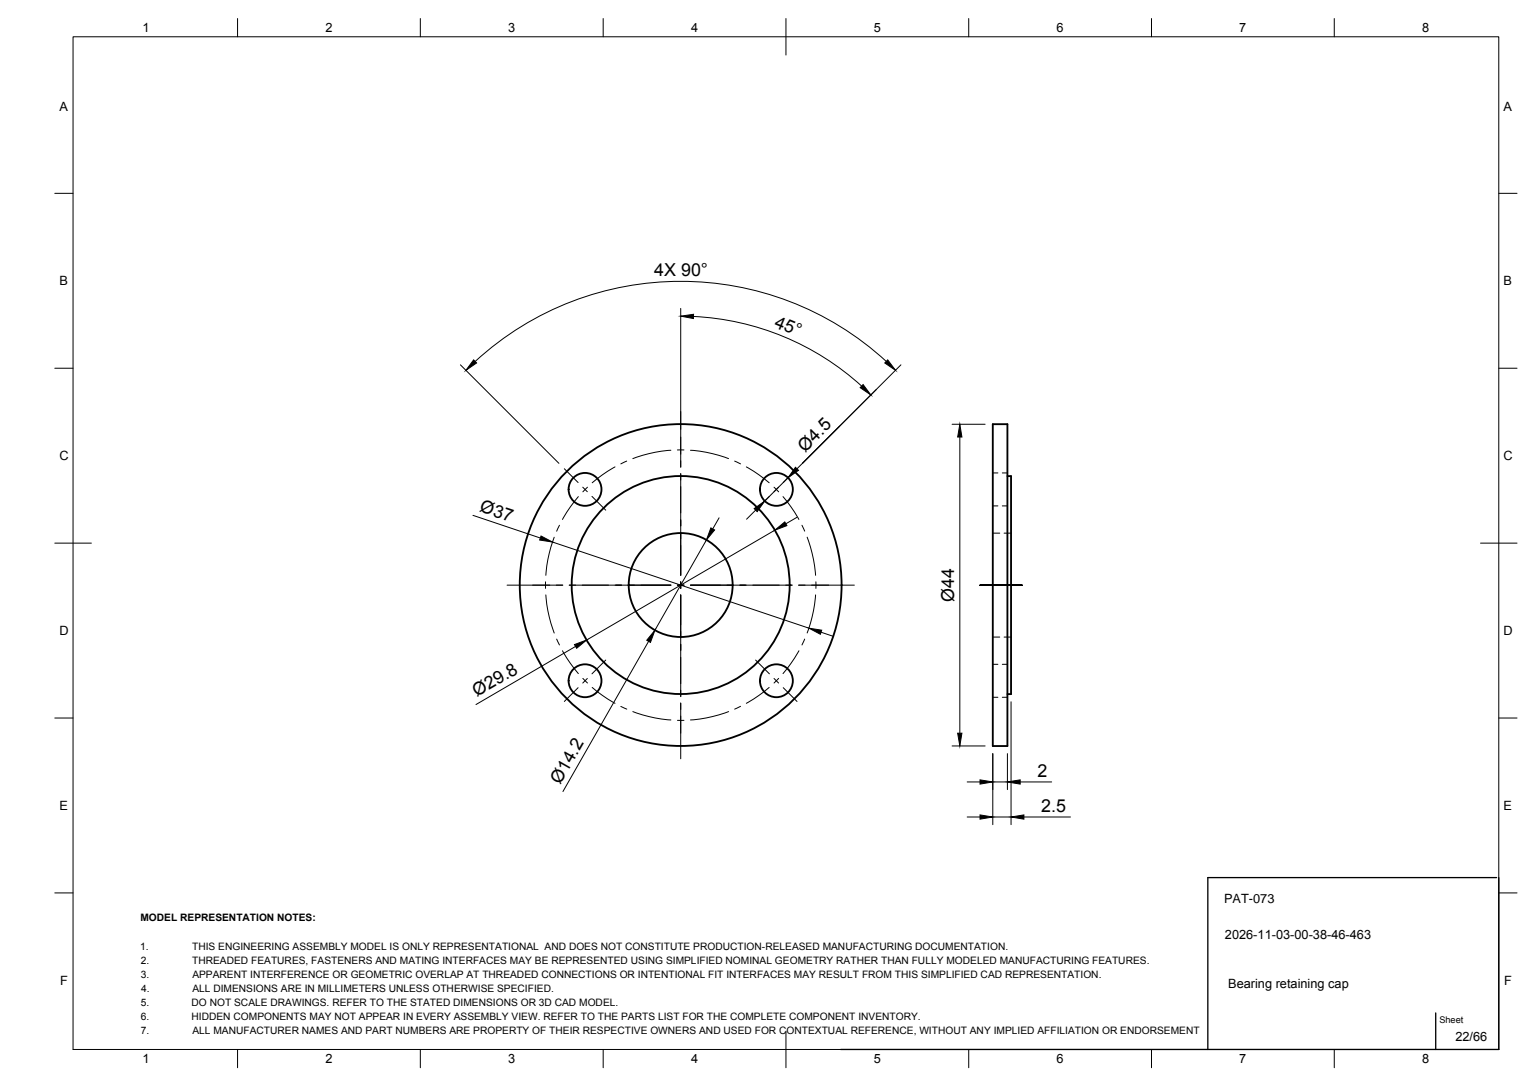
ISO-10303-21;
HEADER;
/* Generated by software containing ST-Developer
 * from STEP Tools, Inc. (www.steptools.com) 
 */

FILE_DESCRIPTION(
/* description */ ('Manual piston pump'),
/* implementation_level */ '2;1');

FILE_NAME(
/* name */ 'Bearing retaining cap.step',
/* time_stamp */ '2026-11-02T16:54:23-08:00',
/* author */ (''),
/* organization */ (''),
/* preprocessor_version */ 'ST-DEVELOPER v20.2',
/* originating_system */ 'Autodesk Translation Framework v15.17.0.0',
/* authorisation */ '');

FILE_SCHEMA (('AUTOMOTIVE_DESIGN { 1 0 10303 214 3 1 1 }'));
ENDSEC;

DATA;
#10=MECHANICAL_DESIGN_GEOMETRIC_PRESENTATION_REPRESENTATION('',(#708),#19043);
#582=SHAPE_REPRESENTATION_RELATIONSHIP('SRR','None',#19328,#645);
#645=ADVANCED_BREP_SHAPE_REPRESENTATION('',(#779),#18995);
#708=STYLED_ITEM('',(#19664),#779);
#779=MANIFOLD_SOLID_BREP('Body1',#9493);
#917=FACE_BOUND('',#2156,.T.);
#918=FACE_BOUND('',#2160,.T.);
#919=FACE_BOUND('',#2161,.T.);
#920=FACE_BOUND('',#2162,.T.);
#921=FACE_BOUND('',#2163,.T.);
#922=FACE_BOUND('',#2164,.T.);
#923=FACE_BOUND('',#2166,.T.);
#924=FACE_BOUND('',#2167,.T.);
#925=FACE_BOUND('',#2168,.T.);
#926=FACE_BOUND('',#2169,.T.);
#927=FACE_BOUND('',#2170,.T.);
#1164=CYLINDRICAL_SURFACE('',#10616,0.225);
#1165=CYLINDRICAL_SURFACE('',#10619,0.225);
#1166=CYLINDRICAL_SURFACE('',#10622,0.225);
#1167=CYLINDRICAL_SURFACE('',#10625,0.225);
#1168=CYLINDRICAL_SURFACE('',#10628,1.49);
#1169=CYLINDRICAL_SURFACE('',#10633,0.710000000000001);
#1170=CYLINDRICAL_SURFACE('',#10635,2.2);
#1485=FACE_OUTER_BOUND('',#2150,.T.);
#1486=FACE_OUTER_BOUND('',#2151,.T.);
#1487=FACE_OUTER_BOUND('',#2152,.T.);
#1488=FACE_OUTER_BOUND('',#2153,.T.);
#1489=FACE_OUTER_BOUND('',#2154,.T.);
#1490=FACE_OUTER_BOUND('',#2155,.T.);
#1491=FACE_OUTER_BOUND('',#2157,.T.);
#1492=FACE_OUTER_BOUND('',#2158,.T.);
#1493=FACE_OUTER_BOUND('',#2159,.T.);
#1494=FACE_OUTER_BOUND('',#2165,.T.);
#2150=EDGE_LOOP('',(#7063,#7064,#7065,#7066));
#2151=EDGE_LOOP('',(#7067,#7068,#7069,#7070));
#2152=EDGE_LOOP('',(#7071,#7072,#7073,#7074));
#2153=EDGE_LOOP('',(#7075,#7076,#7077,#7078));
#2154=EDGE_LOOP('',(#7079,#7080,#7081,#7082));
#2155=EDGE_LOOP('',(#7083));
#2156=EDGE_LOOP('',(#7084));
#2157=EDGE_LOOP('',(#7085,#7086,#7087,#7088));
#2158=EDGE_LOOP('',(#7089,#7090,#7091,#7092));
#2159=EDGE_LOOP('',(#7093));
#2160=EDGE_LOOP('',(#7094));
#2161=EDGE_LOOP('',(#7095));
#2162=EDGE_LOOP('',(#7096));
#2163=EDGE_LOOP('',(#7097));
#2164=EDGE_LOOP('',(#7098));
#2165=EDGE_LOOP('',(#7099));
#2166=EDGE_LOOP('',(#7100));
#2167=EDGE_LOOP('',(#7101));
#2168=EDGE_LOOP('',(#7102));
#2169=EDGE_LOOP('',(#7103));
#2170=EDGE_LOOP('',(#7104));
#2820=CIRCLE('',#10617,0.225);
#2821=CIRCLE('',#10618,0.225);
#2822=CIRCLE('',#10620,0.225);
#2823=CIRCLE('',#10621,0.225);
#2824=CIRCLE('',#10623,0.225);
#2825=CIRCLE('',#10624,0.225);
#2826=CIRCLE('',#10626,0.225);
#2827=CIRCLE('',#10627,0.225);
#2828=CIRCLE('',#10629,1.49);
#2829=CIRCLE('',#10630,1.49);
#2830=CIRCLE('',#10632,0.710000000000001);
#2831=CIRCLE('',#10634,0.710000000000001);
#2832=CIRCLE('',#10636,2.2);
#2833=CIRCLE('',#10637,2.2);
#3370=LINE('',#15553,#3974);
#3371=LINE('',#15559,#3975);
#3372=LINE('',#15565,#3976);
#3373=LINE('',#15571,#3977);
#3374=LINE('',#15577,#3978);
#3375=LINE('',#15584,#3979);
#3376=LINE('',#15590,#3980);
#3974=VECTOR('',#12468,0.225);
#3975=VECTOR('',#12475,0.225);
#3976=VECTOR('',#12482,0.225);
#3977=VECTOR('',#12489,0.225);
#3978=VECTOR('',#12496,1.49);
#3979=VECTOR('',#12505,0.710000000000001);
#3980=VECTOR('',#12512,2.2);
#4615=VERTEX_POINT('',#15550);
#4616=VERTEX_POINT('',#15552);
#4617=VERTEX_POINT('',#15556);
#4618=VERTEX_POINT('',#15558);
#4619=VERTEX_POINT('',#15562);
#4620=VERTEX_POINT('',#15564);
#4621=VERTEX_POINT('',#15568);
#4622=VERTEX_POINT('',#15570);
#4623=VERTEX_POINT('',#15574);
#4624=VERTEX_POINT('',#15576);
#4625=VERTEX_POINT('',#15580);
#4626=VERTEX_POINT('',#15583);
#4627=VERTEX_POINT('',#15587);
#4628=VERTEX_POINT('',#15589);
#5518=EDGE_CURVE('',#4615,#4615,#2820,.T.);
#5519=EDGE_CURVE('',#4615,#4616,#3370,.T.);
#5520=EDGE_CURVE('',#4616,#4616,#2821,.T.);
#5521=EDGE_CURVE('',#4617,#4617,#2822,.T.);
#5522=EDGE_CURVE('',#4617,#4618,#3371,.T.);
#5523=EDGE_CURVE('',#4618,#4618,#2823,.T.);
#5524=EDGE_CURVE('',#4619,#4619,#2824,.T.);
#5525=EDGE_CURVE('',#4619,#4620,#3372,.T.);
#5526=EDGE_CURVE('',#4620,#4620,#2825,.T.);
#5527=EDGE_CURVE('',#4621,#4621,#2826,.T.);
#5528=EDGE_CURVE('',#4621,#4622,#3373,.T.);
#5529=EDGE_CURVE('',#4622,#4622,#2827,.T.);
#5530=EDGE_CURVE('',#4623,#4623,#2828,.T.);
#5531=EDGE_CURVE('',#4623,#4624,#3374,.T.);
#5532=EDGE_CURVE('',#4624,#4624,#2829,.T.);
#5533=EDGE_CURVE('',#4625,#4625,#2830,.T.);
#5534=EDGE_CURVE('',#4625,#4626,#3375,.T.);
#5535=EDGE_CURVE('',#4626,#4626,#2831,.T.);
#5536=EDGE_CURVE('',#4627,#4627,#2832,.T.);
#5537=EDGE_CURVE('',#4627,#4628,#3376,.T.);
#5538=EDGE_CURVE('',#4628,#4628,#2833,.T.);
#7063=ORIENTED_EDGE('',*,*,#5518,.F.);
#7064=ORIENTED_EDGE('',*,*,#5519,.T.);
#7065=ORIENTED_EDGE('',*,*,#5520,.F.);
#7066=ORIENTED_EDGE('',*,*,#5519,.F.);
#7067=ORIENTED_EDGE('',*,*,#5521,.F.);
#7068=ORIENTED_EDGE('',*,*,#5522,.T.);
#7069=ORIENTED_EDGE('',*,*,#5523,.F.);
#7070=ORIENTED_EDGE('',*,*,#5522,.F.);
#7071=ORIENTED_EDGE('',*,*,#5524,.F.);
#7072=ORIENTED_EDGE('',*,*,#5525,.T.);
#7073=ORIENTED_EDGE('',*,*,#5526,.F.);
#7074=ORIENTED_EDGE('',*,*,#5525,.F.);
#7075=ORIENTED_EDGE('',*,*,#5527,.F.);
#7076=ORIENTED_EDGE('',*,*,#5528,.T.);
#7077=ORIENTED_EDGE('',*,*,#5529,.F.);
#7078=ORIENTED_EDGE('',*,*,#5528,.F.);
#7079=ORIENTED_EDGE('',*,*,#5530,.F.);
#7080=ORIENTED_EDGE('',*,*,#5531,.T.);
#7081=ORIENTED_EDGE('',*,*,#5532,.F.);
#7082=ORIENTED_EDGE('',*,*,#5531,.F.);
#7083=ORIENTED_EDGE('',*,*,#5530,.T.);
#7084=ORIENTED_EDGE('',*,*,#5533,.T.);
#7085=ORIENTED_EDGE('',*,*,#5533,.F.);
#7086=ORIENTED_EDGE('',*,*,#5534,.T.);
#7087=ORIENTED_EDGE('',*,*,#5535,.T.);
#7088=ORIENTED_EDGE('',*,*,#5534,.F.);
#7089=ORIENTED_EDGE('',*,*,#5536,.F.);
#7090=ORIENTED_EDGE('',*,*,#5537,.T.);
#7091=ORIENTED_EDGE('',*,*,#5538,.T.);
#7092=ORIENTED_EDGE('',*,*,#5537,.F.);
#7093=ORIENTED_EDGE('',*,*,#5536,.T.);
#7094=ORIENTED_EDGE('',*,*,#5532,.T.);
#7095=ORIENTED_EDGE('',*,*,#5529,.T.);
#7096=ORIENTED_EDGE('',*,*,#5526,.T.);
#7097=ORIENTED_EDGE('',*,*,#5523,.T.);
#7098=ORIENTED_EDGE('',*,*,#5520,.T.);
#7099=ORIENTED_EDGE('',*,*,#5538,.F.);
#7100=ORIENTED_EDGE('',*,*,#5535,.F.);
#7101=ORIENTED_EDGE('',*,*,#5527,.T.);
#7102=ORIENTED_EDGE('',*,*,#5524,.T.);
#7103=ORIENTED_EDGE('',*,*,#5521,.T.);
#7104=ORIENTED_EDGE('',*,*,#5518,.T.);
#8685=PLANE('',#10631);
#8686=PLANE('',#10638);
#8687=PLANE('',#10639);
#9090=ADVANCED_FACE('',(#1485),#1164,.F.);
#9091=ADVANCED_FACE('',(#1486),#1165,.F.);
#9092=ADVANCED_FACE('',(#1487),#1166,.F.);
#9093=ADVANCED_FACE('',(#1488),#1167,.F.);
#9094=ADVANCED_FACE('',(#1489),#1168,.T.);
#9095=ADVANCED_FACE('',(#1490,#917),#8685,.T.);
#9096=ADVANCED_FACE('',(#1491),#1169,.F.);
#9097=ADVANCED_FACE('',(#1492),#1170,.T.);
#9098=ADVANCED_FACE('',(#1493,#918,#919,#920,#921,#922),#8686,.T.);
#9099=ADVANCED_FACE('',(#1494,#923,#924,#925,#926,#927),#8687,.F.);
#9493=CLOSED_SHELL('',(#9090,#9091,#9092,#9093,#9094,#9095,#9096,#9097,
#9098,#9099));
#10615=AXIS2_PLACEMENT_3D('',#15548,#12462,#12463);
#10616=AXIS2_PLACEMENT_3D('',#15549,#12464,#12465);
#10617=AXIS2_PLACEMENT_3D('',#15551,#12466,#12467);
#10618=AXIS2_PLACEMENT_3D('',#15554,#12469,#12470);
#10619=AXIS2_PLACEMENT_3D('',#15555,#12471,#12472);
#10620=AXIS2_PLACEMENT_3D('',#15557,#12473,#12474);
#10621=AXIS2_PLACEMENT_3D('',#15560,#12476,#12477);
#10622=AXIS2_PLACEMENT_3D('',#15561,#12478,#12479);
#10623=AXIS2_PLACEMENT_3D('',#15563,#12480,#12481);
#10624=AXIS2_PLACEMENT_3D('',#15566,#12483,#12484);
#10625=AXIS2_PLACEMENT_3D('',#15567,#12485,#12486);
#10626=AXIS2_PLACEMENT_3D('',#15569,#12487,#12488);
#10627=AXIS2_PLACEMENT_3D('',#15572,#12490,#12491);
#10628=AXIS2_PLACEMENT_3D('',#15573,#12492,#12493);
#10629=AXIS2_PLACEMENT_3D('',#15575,#12494,#12495);
#10630=AXIS2_PLACEMENT_3D('',#15578,#12497,#12498);
#10631=AXIS2_PLACEMENT_3D('',#15579,#12499,#12500);
#10632=AXIS2_PLACEMENT_3D('',#15581,#12501,#12502);
#10633=AXIS2_PLACEMENT_3D('',#15582,#12503,#12504);
#10634=AXIS2_PLACEMENT_3D('',#15585,#12506,#12507);
#10635=AXIS2_PLACEMENT_3D('',#15586,#12508,#12509);
#10636=AXIS2_PLACEMENT_3D('',#15588,#12510,#12511);
#10637=AXIS2_PLACEMENT_3D('',#15591,#12513,#12514);
#10638=AXIS2_PLACEMENT_3D('',#15592,#12515,#12516);
#10639=AXIS2_PLACEMENT_3D('',#15593,#12517,#12518);
#12462=DIRECTION('axis',(0.,0.,1.));
#12463=DIRECTION('refdir',(1.,0.,0.));
#12464=DIRECTION('center_axis',(1.,0.,0.));
#12465=DIRECTION('ref_axis',(0.,0.,-1.));
#12466=DIRECTION('center_axis',(1.,0.,0.));
#12467=DIRECTION('ref_axis',(0.,0.,-1.));
#12468=DIRECTION('',(1.,0.,0.));
#12469=DIRECTION('center_axis',(-1.,0.,0.));
#12470=DIRECTION('ref_axis',(0.,0.,-1.));
#12471=DIRECTION('center_axis',(1.,0.,0.));
#12472=DIRECTION('ref_axis',(0.,0.,-1.));
#12473=DIRECTION('center_axis',(1.,0.,0.));
#12474=DIRECTION('ref_axis',(0.,0.,-1.));
#12475=DIRECTION('',(1.,0.,0.));
#12476=DIRECTION('center_axis',(-1.,0.,0.));
#12477=DIRECTION('ref_axis',(0.,0.,-1.));
#12478=DIRECTION('center_axis',(1.,0.,0.));
#12479=DIRECTION('ref_axis',(0.,0.,-1.));
#12480=DIRECTION('center_axis',(1.,0.,0.));
#12481=DIRECTION('ref_axis',(0.,0.,-1.));
#12482=DIRECTION('',(1.,0.,0.));
#12483=DIRECTION('center_axis',(-1.,0.,0.));
#12484=DIRECTION('ref_axis',(0.,0.,-1.));
#12485=DIRECTION('center_axis',(1.,0.,0.));
#12486=DIRECTION('ref_axis',(0.,0.,-1.));
#12487=DIRECTION('center_axis',(1.,0.,0.));
#12488=DIRECTION('ref_axis',(0.,0.,-1.));
#12489=DIRECTION('',(1.,0.,0.));
#12490=DIRECTION('center_axis',(-1.,0.,0.));
#12491=DIRECTION('ref_axis',(0.,0.,-1.));
#12492=DIRECTION('center_axis',(1.,0.,0.));
#12493=DIRECTION('ref_axis',(0.,0.,-1.));
#12494=DIRECTION('center_axis',(1.,0.,0.));
#12495=DIRECTION('ref_axis',(0.,0.,-1.));
#12496=DIRECTION('',(-1.,0.,0.));
#12497=DIRECTION('center_axis',(-1.,0.,0.));
#12498=DIRECTION('ref_axis',(0.,0.,-1.));
#12499=DIRECTION('center_axis',(1.,0.,0.));
#12500=DIRECTION('ref_axis',(0.,0.,-1.));
#12501=DIRECTION('center_axis',(-1.,0.,0.));
#12502=DIRECTION('ref_axis',(0.,0.,-1.));
#12503=DIRECTION('center_axis',(1.,0.,0.));
#12504=DIRECTION('ref_axis',(0.,0.,-1.));
#12505=DIRECTION('',(-1.,0.,0.));
#12506=DIRECTION('center_axis',(-1.,0.,0.));
#12507=DIRECTION('ref_axis',(0.,0.,-1.));
#12508=DIRECTION('center_axis',(1.,0.,0.));
#12509=DIRECTION('ref_axis',(0.,0.,-1.));
#12510=DIRECTION('center_axis',(1.,0.,0.));
#12511=DIRECTION('ref_axis',(0.,0.,-1.));
#12512=DIRECTION('',(-1.,0.,0.));
#12513=DIRECTION('center_axis',(1.,0.,0.));
#12514=DIRECTION('ref_axis',(0.,0.,-1.));
#12515=DIRECTION('center_axis',(1.,0.,0.));
#12516=DIRECTION('ref_axis',(0.,0.,-1.));
#12517=DIRECTION('center_axis',(1.,0.,0.));
#12518=DIRECTION('ref_axis',(0.,0.,-1.));
#15548=CARTESIAN_POINT('',(0.,0.,0.));
#15549=CARTESIAN_POINT('Origin',(-3.3,-5.30814754519511,8.69185245480489));
#15550=CARTESIAN_POINT('',(-3.2,-5.30814754519511,8.91685245480489));
#15551=CARTESIAN_POINT('Origin',(-3.2,-5.30814754519511,8.69185245480489));
#15552=CARTESIAN_POINT('',(-3.,-5.30814754519511,8.91685245480489));
#15553=CARTESIAN_POINT('',(-3.3,-5.30814754519511,8.91685245480489));
#15554=CARTESIAN_POINT('Origin',(-3.,-5.30814754519511,8.69185245480489));
#15555=CARTESIAN_POINT('Origin',(-3.3,-5.30814754519511,11.3081475451951));
#15556=CARTESIAN_POINT('',(-3.2,-5.30814754519511,11.5331475451951));
#15557=CARTESIAN_POINT('Origin',(-3.2,-5.30814754519511,11.3081475451951));
#15558=CARTESIAN_POINT('',(-3.,-5.30814754519511,11.5331475451951));
#15559=CARTESIAN_POINT('',(-3.3,-5.30814754519511,11.5331475451951));
#15560=CARTESIAN_POINT('Origin',(-3.,-5.30814754519511,11.3081475451951));
#15561=CARTESIAN_POINT('Origin',(-3.3,-2.69185245480489,11.3081475451951));
#15562=CARTESIAN_POINT('',(-3.2,-2.69185245480489,11.5331475451951));
#15563=CARTESIAN_POINT('Origin',(-3.2,-2.69185245480489,11.3081475451951));
#15564=CARTESIAN_POINT('',(-3.,-2.69185245480489,11.5331475451951));
#15565=CARTESIAN_POINT('',(-3.3,-2.69185245480489,11.5331475451951));
#15566=CARTESIAN_POINT('Origin',(-3.,-2.69185245480489,11.3081475451951));
#15567=CARTESIAN_POINT('Origin',(-3.3,-2.69185245480489,8.69185245480489));
#15568=CARTESIAN_POINT('',(-3.2,-2.69185245480489,8.91685245480489));
#15569=CARTESIAN_POINT('Origin',(-3.2,-2.69185245480489,8.69185245480489));
#15570=CARTESIAN_POINT('',(-3.,-2.69185245480489,8.91685245480489));
#15571=CARTESIAN_POINT('',(-3.3,-2.69185245480489,8.91685245480489));
#15572=CARTESIAN_POINT('Origin',(-3.,-2.69185245480489,8.69185245480489));
#15573=CARTESIAN_POINT('Origin',(-3.,-4.,10.));
#15574=CARTESIAN_POINT('',(-2.95,-4.,11.49));
#15575=CARTESIAN_POINT('Origin',(-2.95,-4.,10.));
#15576=CARTESIAN_POINT('',(-3.,-4.,11.49));
#15577=CARTESIAN_POINT('',(-3.,-4.,11.49));
#15578=CARTESIAN_POINT('Origin',(-3.,-4.,10.));
#15579=CARTESIAN_POINT('Origin',(-2.95,-4.,10.));
#15580=CARTESIAN_POINT('',(-2.95,-4.,10.71));
#15581=CARTESIAN_POINT('Origin',(-2.95,-4.,10.));
#15582=CARTESIAN_POINT('Origin',(-3.2,-4.,10.));
#15583=CARTESIAN_POINT('',(-3.2,-4.,10.71));
#15584=CARTESIAN_POINT('',(-3.2,-4.,10.71));
#15585=CARTESIAN_POINT('Origin',(-3.2,-4.,10.));
#15586=CARTESIAN_POINT('Origin',(-3.2,-4.,10.));
#15587=CARTESIAN_POINT('',(-3.,-4.,12.2));
#15588=CARTESIAN_POINT('Origin',(-3.,-4.,10.));
#15589=CARTESIAN_POINT('',(-3.2,-4.,12.2));
#15590=CARTESIAN_POINT('',(-3.2,-4.,12.2));
#15591=CARTESIAN_POINT('Origin',(-3.2,-4.,10.));
#15592=CARTESIAN_POINT('Origin',(-3.,-4.,10.));
#15593=CARTESIAN_POINT('Origin',(-3.2,-4.,10.));
#18924=UNCERTAINTY_MEASURE_WITH_UNIT(LENGTH_MEASURE(0.001),#19044,
'DISTANCE_ACCURACY_VALUE',
'Maximum model space distance between geometric entities at asserted c
onnectivities');
#18972=UNCERTAINTY_MEASURE_WITH_UNIT(LENGTH_MEASURE(0.001),#19044,
'DISTANCE_ACCURACY_VALUE',
'Maximum model space distance between geometric entities at asserted c
onnectivities');
#18995=(
GEOMETRIC_REPRESENTATION_CONTEXT(3)
GLOBAL_UNCERTAINTY_ASSIGNED_CONTEXT((#18924))
GLOBAL_UNIT_ASSIGNED_CONTEXT((#19044,#19046,#19047))
REPRESENTATION_CONTEXT('','3D')
);
#19043=(
GEOMETRIC_REPRESENTATION_CONTEXT(3)
GLOBAL_UNCERTAINTY_ASSIGNED_CONTEXT((#18972))
GLOBAL_UNIT_ASSIGNED_CONTEXT((#19044,#19046,#19047))
REPRESENTATION_CONTEXT('','3D')
);
#19044=(
LENGTH_UNIT()
NAMED_UNIT(*)
SI_UNIT(.CENTI.,.METRE.)
);
#19046=(
NAMED_UNIT(*)
PLANE_ANGLE_UNIT()
SI_UNIT($,.RADIAN.)
);
#19047=(
NAMED_UNIT(*)
SI_UNIT($,.STERADIAN.)
SOLID_ANGLE_UNIT()
);
#19070=SHAPE_DEFINITION_REPRESENTATION(#19140,#19328);
#19140=PRODUCT_DEFINITION_SHAPE('',$,#19399);
#19328=SHAPE_REPRESENTATION('',(#10615),#18995);
#19376=PRODUCT_DEFINITION_CONTEXT('part definition',#19588,'design');
#19399=PRODUCT_DEFINITION('2026-11-03-00-38-46-463',
'Bearing retaining cap',#19469,#19376);
#19469=PRODUCT_DEFINITION_FORMATION('',$,#19612);
#19588=APPLICATION_CONTEXT(
'Core Data for Automotive Mechanical Design Process');
#19589=PRODUCT_CONTEXT('part definition',#19588,'mechanical');
#19612=PRODUCT('2026-11-03-00-38-46-463','Bearing retaining cap',
'Bearing retaining cap',(#19589));
#19664=PRESENTATION_STYLE_ASSIGNMENT((#19670));
#19670=SURFACE_STYLE_USAGE(.BOTH.,#19676);
#19676=SURFACE_SIDE_STYLE('',(#19682));
#19682=SURFACE_STYLE_FILL_AREA(#19688);
#19688=FILL_AREA_STYLE('CAD Library Painted - Steel gray',(#19694));
#19694=FILL_AREA_STYLE_COLOUR('CAD Library Painted - Steel gray',#19700);
#19700=COLOUR_RGB('CAD Library Painted - Steel gray',0.592156862745098,
0.631372549019608,0.67843137254902);
ENDSEC;
END-ISO-10303-21;
